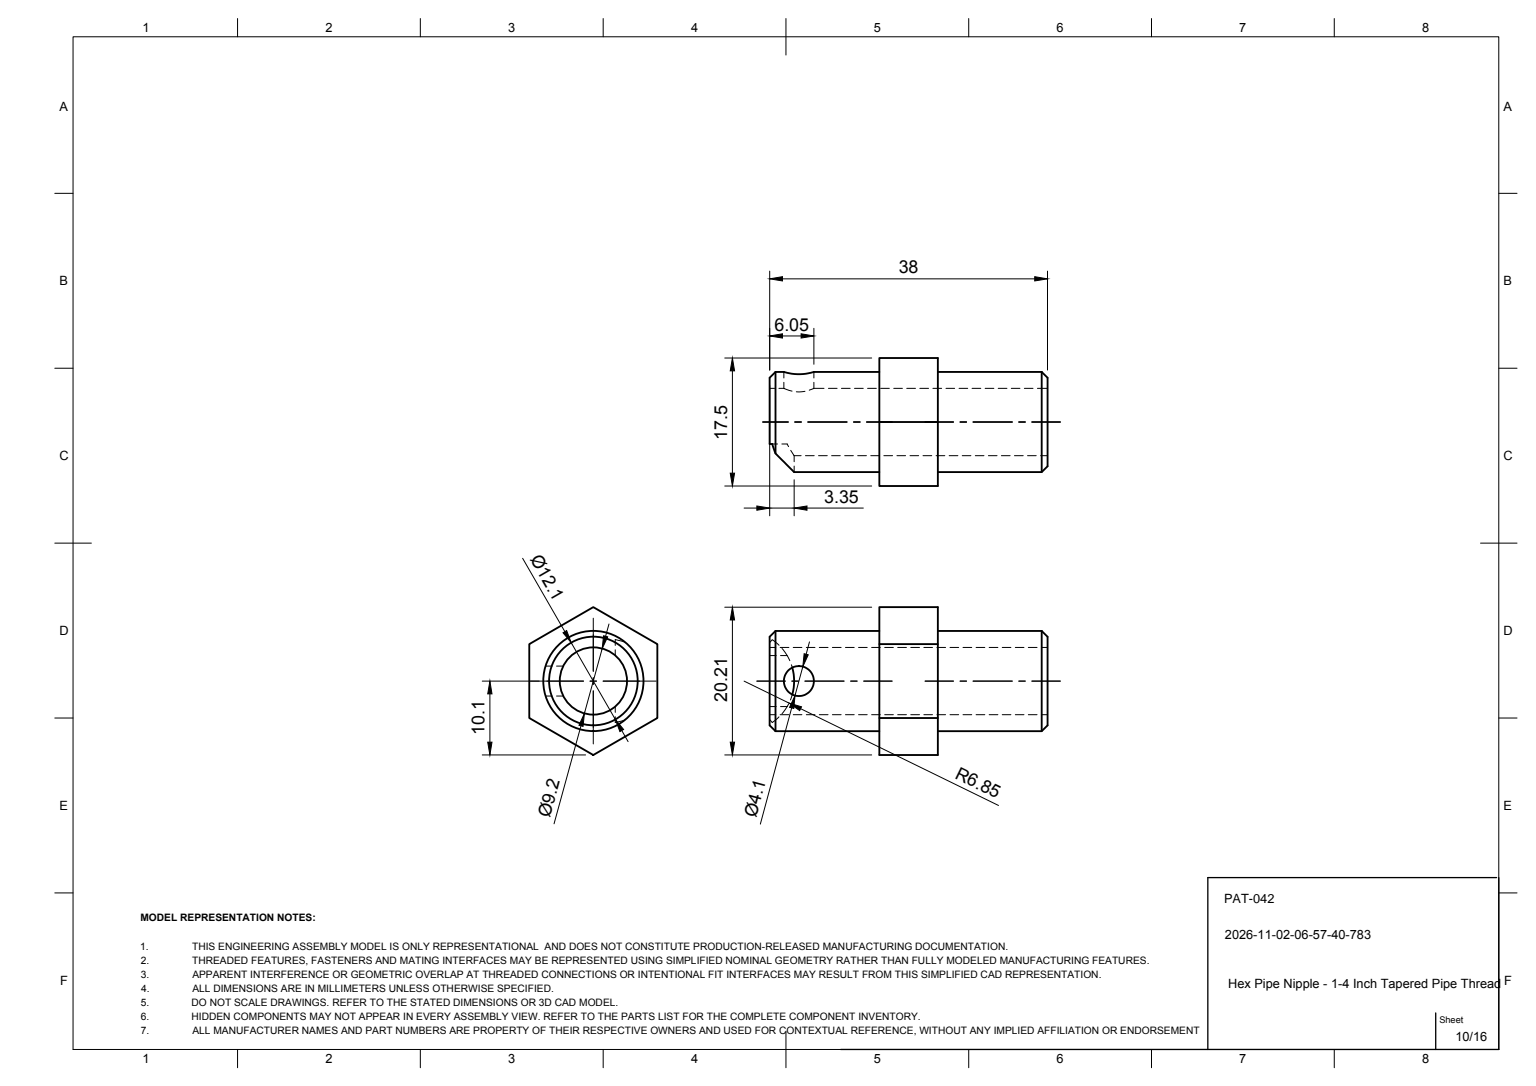
ISO-10303-21;
HEADER;
/* Generated by software containing ST-Developer
 * from STEP Tools, Inc. (www.steptools.com) 
 */

FILE_DESCRIPTION(
/* description */ ('Manifold and mounting hardware'),
/* implementation_level */ '2;1');

FILE_NAME(
/* name */ 'Hex Pipe Nipple - 1-4 Inch Tapered Pipe Thread.step',
/* time_stamp */ '2026-10-28T21:46:49-07:00',
/* author */ (''),
/* organization */ (''),
/* preprocessor_version */ 'ST-DEVELOPER v20.2',
/* originating_system */ 'Autodesk Translation Framework v15.17.0.0',
/* authorisation */ '');

FILE_SCHEMA (('AUTOMOTIVE_DESIGN { 1 0 10303 214 3 1 1 }'));
ENDSEC;

DATA;
#10=MECHANICAL_DESIGN_GEOMETRIC_PRESENTATION_REPRESENTATION('',(#157),#5638);
#118=CONICAL_SURFACE('',#3555,0.645,0.785398163397448);
#129=SHAPE_REPRESENTATION_RELATIONSHIP('SRR','None',#5708,#143);
#143=ADVANCED_BREP_SHAPE_REPRESENTATION('',(#171),#5630);
#157=STYLED_ITEM('',(#5853),#171);
#171=MANIFOLD_SOLID_BREP('Body1',#3147);
#236=FACE_BOUND('',#694,.T.);
#237=FACE_BOUND('',#697,.T.);
#238=FACE_BOUND('',#699,.T.);
#239=FACE_BOUND('',#710,.T.);
#314=CYLINDRICAL_SURFACE('',#3540,0.46);
#315=CYLINDRICAL_SURFACE('',#3552,0.685);
#316=CYLINDRICAL_SURFACE('',#3553,0.685);
#449=FACE_OUTER_BOUND('',#693,.T.);
#450=FACE_OUTER_BOUND('',#695,.T.);
#451=FACE_OUTER_BOUND('',#696,.T.);
#452=FACE_OUTER_BOUND('',#698,.T.);
#453=FACE_OUTER_BOUND('',#700,.T.);
#454=FACE_OUTER_BOUND('',#701,.T.);
#455=FACE_OUTER_BOUND('',#702,.T.);
#456=FACE_OUTER_BOUND('',#703,.T.);
#457=FACE_OUTER_BOUND('',#704,.T.);
#458=FACE_OUTER_BOUND('',#705,.T.);
#459=FACE_OUTER_BOUND('',#706,.T.);
#460=FACE_OUTER_BOUND('',#707,.T.);
#461=FACE_OUTER_BOUND('',#708,.T.);
#462=FACE_OUTER_BOUND('',#709,.T.);
#693=EDGE_LOOP('',(#2574));
#694=EDGE_LOOP('',(#2575));
#695=EDGE_LOOP('',(#2576,#2577,#2578,#2579));
#696=EDGE_LOOP('',(#2580,#2581,#2582,#2583,#2584,#2585));
#697=EDGE_LOOP('',(#2586));
#698=EDGE_LOOP('',(#2587,#2588,#2589,#2590,#2591,#2592));
#699=EDGE_LOOP('',(#2593));
#700=EDGE_LOOP('',(#2594,#2595,#2596,#2597));
#701=EDGE_LOOP('',(#2598,#2599,#2600,#2601));
#702=EDGE_LOOP('',(#2602,#2603,#2604,#2605));
#703=EDGE_LOOP('',(#2606,#2607,#2608,#2609));
#704=EDGE_LOOP('',(#2610,#2611,#2612,#2613));
#705=EDGE_LOOP('',(#2614,#2615,#2616,#2617));
#706=EDGE_LOOP('',(#2618,#2619,#2620,#2621));
#707=EDGE_LOOP('',(#2622,#2623,#2624,#2625));
#708=EDGE_LOOP('',(#2626,#2627,#2628,#2629));
#709=EDGE_LOOP('',(#2630));
#710=EDGE_LOOP('',(#2631));
#861=CIRCLE('',#3538,0.685);
#862=CIRCLE('',#3539,0.46);
#863=CIRCLE('',#3541,0.46);
#864=CIRCLE('',#3543,0.685);
#865=CIRCLE('',#3545,0.685);
#866=CIRCLE('',#3554,0.685);
#867=CIRCLE('',#3556,0.605);
#1058=LINE('',#5290,#1305);
#1059=LINE('',#5294,#1306);
#1060=LINE('',#5296,#1307);
#1061=LINE('',#5298,#1308);
#1062=LINE('',#5300,#1309);
#1063=LINE('',#5302,#1310);
#1064=LINE('',#5303,#1311);
#1065=LINE('',#5309,#1312);
#1066=LINE('',#5311,#1313);
#1067=LINE('',#5313,#1314);
#1068=LINE('',#5315,#1315);
#1069=LINE('',#5317,#1316);
#1070=LINE('',#5318,#1317);
#1071=LINE('',#5322,#1318);
#1072=LINE('',#5323,#1319);
#1073=LINE('',#5325,#1320);
#1074=LINE('',#5327,#1321);
#1075=LINE('',#5329,#1322);
#1076=LINE('',#5331,#1323);
#1077=LINE('',#5334,#1324);
#1078=LINE('',#5338,#1325);
#1079=LINE('',#5342,#1326);
#1305=VECTOR('',#4299,0.46);
#1306=VECTOR('',#4302,1.);
#1307=VECTOR('',#4303,1.);
#1308=VECTOR('',#4304,1.);
#1309=VECTOR('',#4305,1.);
#1310=VECTOR('',#4306,1.);
#1311=VECTOR('',#4307,1.);
#1312=VECTOR('',#4312,1.);
#1313=VECTOR('',#4313,1.);
#1314=VECTOR('',#4314,1.);
#1315=VECTOR('',#4315,1.);
#1316=VECTOR('',#4316,1.);
#1317=VECTOR('',#4317,1.);
#1318=VECTOR('',#4322,1.);
#1319=VECTOR('',#4323,1.);
#1320=VECTOR('',#4326,1.);
#1321=VECTOR('',#4329,1.);
#1322=VECTOR('',#4332,1.);
#1323=VECTOR('',#4335,1.);
#1324=VECTOR('',#4340,0.685);
#1325=VECTOR('',#4345,0.685);
#1326=VECTOR('',#4350,0.645);
#1567=VERTEX_POINT('',#5283);
#1568=VERTEX_POINT('',#5285);
#1569=VERTEX_POINT('',#5288);
#1570=VERTEX_POINT('',#5292);
#1571=VERTEX_POINT('',#5293);
#1572=VERTEX_POINT('',#5295);
#1573=VERTEX_POINT('',#5297);
#1574=VERTEX_POINT('',#5299);
#1575=VERTEX_POINT('',#5301);
#1576=VERTEX_POINT('',#5304);
#1577=VERTEX_POINT('',#5307);
#1578=VERTEX_POINT('',#5308);
#1579=VERTEX_POINT('',#5310);
#1580=VERTEX_POINT('',#5312);
#1581=VERTEX_POINT('',#5314);
#1582=VERTEX_POINT('',#5316);
#1583=VERTEX_POINT('',#5319);
#1584=VERTEX_POINT('',#5336);
#1585=VERTEX_POINT('',#5340);
#1916=EDGE_CURVE('',#1567,#1567,#861,.T.);
#1917=EDGE_CURVE('',#1568,#1568,#862,.T.);
#1918=EDGE_CURVE('',#1569,#1569,#863,.T.);
#1919=EDGE_CURVE('',#1569,#1568,#1058,.T.);
#1920=EDGE_CURVE('',#1570,#1571,#1059,.T.);
#1921=EDGE_CURVE('',#1571,#1572,#1060,.T.);
#1922=EDGE_CURVE('',#1572,#1573,#1061,.T.);
#1923=EDGE_CURVE('',#1573,#1574,#1062,.T.);
#1924=EDGE_CURVE('',#1574,#1575,#1063,.T.);
#1925=EDGE_CURVE('',#1575,#1570,#1064,.T.);
#1926=EDGE_CURVE('',#1576,#1576,#864,.T.);
#1927=EDGE_CURVE('',#1577,#1578,#1065,.T.);
#1928=EDGE_CURVE('',#1578,#1579,#1066,.T.);
#1929=EDGE_CURVE('',#1579,#1580,#1067,.T.);
#1930=EDGE_CURVE('',#1580,#1581,#1068,.T.);
#1931=EDGE_CURVE('',#1581,#1582,#1069,.T.);
#1932=EDGE_CURVE('',#1582,#1577,#1070,.T.);
#1933=EDGE_CURVE('',#1583,#1583,#865,.T.);
#1934=EDGE_CURVE('',#1577,#1571,#1071,.T.);
#1935=EDGE_CURVE('',#1572,#1582,#1072,.T.);
#1936=EDGE_CURVE('',#1573,#1581,#1073,.T.);
#1937=EDGE_CURVE('',#1574,#1580,#1074,.T.);
#1938=EDGE_CURVE('',#1575,#1579,#1075,.T.);
#1939=EDGE_CURVE('',#1570,#1578,#1076,.T.);
#1940=EDGE_CURVE('',#1583,#1567,#1077,.T.);
#1941=EDGE_CURVE('',#1584,#1584,#866,.T.);
#1942=EDGE_CURVE('',#1584,#1576,#1078,.T.);
#1943=EDGE_CURVE('',#1585,#1585,#867,.T.);
#1944=EDGE_CURVE('',#1585,#1584,#1079,.T.);
#2574=ORIENTED_EDGE('',*,*,#1916,.F.);
#2575=ORIENTED_EDGE('',*,*,#1917,.F.);
#2576=ORIENTED_EDGE('',*,*,#1918,.T.);
#2577=ORIENTED_EDGE('',*,*,#1919,.T.);
#2578=ORIENTED_EDGE('',*,*,#1917,.T.);
#2579=ORIENTED_EDGE('',*,*,#1919,.F.);
#2580=ORIENTED_EDGE('',*,*,#1920,.T.);
#2581=ORIENTED_EDGE('',*,*,#1921,.T.);
#2582=ORIENTED_EDGE('',*,*,#1922,.T.);
#2583=ORIENTED_EDGE('',*,*,#1923,.T.);
#2584=ORIENTED_EDGE('',*,*,#1924,.T.);
#2585=ORIENTED_EDGE('',*,*,#1925,.T.);
#2586=ORIENTED_EDGE('',*,*,#1926,.F.);
#2587=ORIENTED_EDGE('',*,*,#1927,.T.);
#2588=ORIENTED_EDGE('',*,*,#1928,.T.);
#2589=ORIENTED_EDGE('',*,*,#1929,.T.);
#2590=ORIENTED_EDGE('',*,*,#1930,.T.);
#2591=ORIENTED_EDGE('',*,*,#1931,.T.);
#2592=ORIENTED_EDGE('',*,*,#1932,.T.);
#2593=ORIENTED_EDGE('',*,*,#1933,.F.);
#2594=ORIENTED_EDGE('',*,*,#1934,.F.);
#2595=ORIENTED_EDGE('',*,*,#1932,.F.);
#2596=ORIENTED_EDGE('',*,*,#1935,.F.);
#2597=ORIENTED_EDGE('',*,*,#1921,.F.);
#2598=ORIENTED_EDGE('',*,*,#1935,.T.);
#2599=ORIENTED_EDGE('',*,*,#1931,.F.);
#2600=ORIENTED_EDGE('',*,*,#1936,.F.);
#2601=ORIENTED_EDGE('',*,*,#1922,.F.);
#2602=ORIENTED_EDGE('',*,*,#1936,.T.);
#2603=ORIENTED_EDGE('',*,*,#1930,.F.);
#2604=ORIENTED_EDGE('',*,*,#1937,.F.);
#2605=ORIENTED_EDGE('',*,*,#1923,.F.);
#2606=ORIENTED_EDGE('',*,*,#1937,.T.);
#2607=ORIENTED_EDGE('',*,*,#1929,.F.);
#2608=ORIENTED_EDGE('',*,*,#1938,.F.);
#2609=ORIENTED_EDGE('',*,*,#1924,.F.);
#2610=ORIENTED_EDGE('',*,*,#1938,.T.);
#2611=ORIENTED_EDGE('',*,*,#1928,.F.);
#2612=ORIENTED_EDGE('',*,*,#1939,.F.);
#2613=ORIENTED_EDGE('',*,*,#1925,.F.);
#2614=ORIENTED_EDGE('',*,*,#1939,.T.);
#2615=ORIENTED_EDGE('',*,*,#1927,.F.);
#2616=ORIENTED_EDGE('',*,*,#1934,.T.);
#2617=ORIENTED_EDGE('',*,*,#1920,.F.);
#2618=ORIENTED_EDGE('',*,*,#1933,.T.);
#2619=ORIENTED_EDGE('',*,*,#1940,.T.);
#2620=ORIENTED_EDGE('',*,*,#1916,.T.);
#2621=ORIENTED_EDGE('',*,*,#1940,.F.);
#2622=ORIENTED_EDGE('',*,*,#1941,.F.);
#2623=ORIENTED_EDGE('',*,*,#1942,.T.);
#2624=ORIENTED_EDGE('',*,*,#1926,.T.);
#2625=ORIENTED_EDGE('',*,*,#1942,.F.);
#2626=ORIENTED_EDGE('',*,*,#1943,.F.);
#2627=ORIENTED_EDGE('',*,*,#1944,.T.);
#2628=ORIENTED_EDGE('',*,*,#1941,.T.);
#2629=ORIENTED_EDGE('',*,*,#1944,.F.);
#2630=ORIENTED_EDGE('',*,*,#1943,.T.);
#2631=ORIENTED_EDGE('',*,*,#1918,.F.);
#2908=PLANE('',#3537);
#2909=PLANE('',#3542);
#2910=PLANE('',#3544);
#2911=PLANE('',#3546);
#2912=PLANE('',#3547);
#2913=PLANE('',#3548);
#2914=PLANE('',#3549);
#2915=PLANE('',#3550);
#2916=PLANE('',#3551);
#2917=PLANE('',#3557);
#3073=ADVANCED_FACE('',(#449,#236),#2908,.T.);
#3074=ADVANCED_FACE('',(#450),#314,.F.);
#3075=ADVANCED_FACE('',(#451,#237),#2909,.F.);
#3076=ADVANCED_FACE('',(#452,#238),#2910,.T.);
#3077=ADVANCED_FACE('',(#453),#2911,.T.);
#3078=ADVANCED_FACE('',(#454),#2912,.T.);
#3079=ADVANCED_FACE('',(#455),#2913,.T.);
#3080=ADVANCED_FACE('',(#456),#2914,.T.);
#3081=ADVANCED_FACE('',(#457),#2915,.T.);
#3082=ADVANCED_FACE('',(#458),#2916,.T.);
#3083=ADVANCED_FACE('',(#459),#315,.T.);
#3084=ADVANCED_FACE('',(#460),#316,.T.);
#3085=ADVANCED_FACE('',(#461),#118,.T.);
#3086=ADVANCED_FACE('',(#462,#239),#2917,.T.);
#3147=CLOSED_SHELL('',(#3073,#3074,#3075,#3076,#3077,#3078,#3079,#3080,
#3081,#3082,#3083,#3084,#3085,#3086));
#3536=AXIS2_PLACEMENT_3D('',#5281,#4287,#4288);
#3537=AXIS2_PLACEMENT_3D('',#5282,#4289,#4290);
#3538=AXIS2_PLACEMENT_3D('',#5284,#4291,#4292);
#3539=AXIS2_PLACEMENT_3D('',#5286,#4293,#4294);
#3540=AXIS2_PLACEMENT_3D('',#5287,#4295,#4296);
#3541=AXIS2_PLACEMENT_3D('',#5289,#4297,#4298);
#3542=AXIS2_PLACEMENT_3D('',#5291,#4300,#4301);
#3543=AXIS2_PLACEMENT_3D('',#5305,#4308,#4309);
#3544=AXIS2_PLACEMENT_3D('',#5306,#4310,#4311);
#3545=AXIS2_PLACEMENT_3D('',#5320,#4318,#4319);
#3546=AXIS2_PLACEMENT_3D('',#5321,#4320,#4321);
#3547=AXIS2_PLACEMENT_3D('',#5324,#4324,#4325);
#3548=AXIS2_PLACEMENT_3D('',#5326,#4327,#4328);
#3549=AXIS2_PLACEMENT_3D('',#5328,#4330,#4331);
#3550=AXIS2_PLACEMENT_3D('',#5330,#4333,#4334);
#3551=AXIS2_PLACEMENT_3D('',#5332,#4336,#4337);
#3552=AXIS2_PLACEMENT_3D('',#5333,#4338,#4339);
#3553=AXIS2_PLACEMENT_3D('',#5335,#4341,#4342);
#3554=AXIS2_PLACEMENT_3D('',#5337,#4343,#4344);
#3555=AXIS2_PLACEMENT_3D('',#5339,#4346,#4347);
#3556=AXIS2_PLACEMENT_3D('',#5341,#4348,#4349);
#3557=AXIS2_PLACEMENT_3D('',#5343,#4351,#4352);
#4287=DIRECTION('axis',(0.,0.,1.));
#4288=DIRECTION('refdir',(1.,0.,0.));
#4289=DIRECTION('center_axis',(1.14015052621434E-31,1.,-1.55447022770527E-24));
#4290=DIRECTION('ref_axis',(-1.,1.10933564796705E-31,5.55111512312579E-17));
#4291=DIRECTION('center_axis',(-1.14015052621434E-31,-1.,1.55447022770527E-24));
#4292=DIRECTION('ref_axis',(1.,0.,0.));
#4293=DIRECTION('center_axis',(1.14015052621434E-31,1.,-1.55447022770527E-24));
#4294=DIRECTION('ref_axis',(1.,0.,0.));
#4295=DIRECTION('center_axis',(0.,-1.,0.));
#4296=DIRECTION('ref_axis',(1.,0.,0.));
#4297=DIRECTION('center_axis',(0.,-1.,0.));
#4298=DIRECTION('ref_axis',(1.,0.,0.));
#4299=DIRECTION('',(0.,1.,0.));
#4300=DIRECTION('center_axis',(0.,1.,0.));
#4301=DIRECTION('ref_axis',(1.,0.,0.));
#4302=DIRECTION('',(-0.5,0.,0.866025403784439));
#4303=DIRECTION('',(-1.,0.,-3.29650746237182E-16));
#4304=DIRECTION('',(-0.5,0.,-0.866025403784439));
#4305=DIRECTION('',(0.5,0.,-0.866025403784438));
#4306=DIRECTION('',(1.,0.,0.));
#4307=DIRECTION('',(0.5,0.,0.866025403784439));
#4308=DIRECTION('center_axis',(0.,-1.,0.));
#4309=DIRECTION('ref_axis',(1.,0.,0.));
#4310=DIRECTION('center_axis',(0.,1.,0.));
#4311=DIRECTION('ref_axis',(1.,0.,0.));
#4312=DIRECTION('',(0.5,0.,-0.866025403784439));
#4313=DIRECTION('',(-0.5,0.,-0.866025403784439));
#4314=DIRECTION('',(-1.,0.,0.));
#4315=DIRECTION('',(-0.5,0.,0.866025403784438));
#4316=DIRECTION('',(0.5,0.,0.866025403784439));
#4317=DIRECTION('',(1.,0.,3.29650746237182E-16));
#4318=DIRECTION('center_axis',(0.,1.,0.));
#4319=DIRECTION('ref_axis',(1.,0.,0.));
#4320=DIRECTION('center_axis',(-3.29650746237182E-16,0.,1.));
#4321=DIRECTION('ref_axis',(1.,0.,3.29650746237182E-16));
#4322=DIRECTION('',(0.,-1.,0.));
#4323=DIRECTION('',(0.,1.,0.));
#4324=DIRECTION('center_axis',(-0.866025403784439,0.,0.5));
#4325=DIRECTION('ref_axis',(0.5,0.,0.866025403784439));
#4326=DIRECTION('',(0.,1.,0.));
#4327=DIRECTION('center_axis',(-0.866025403784439,0.,-0.5));
#4328=DIRECTION('ref_axis',(-0.5,0.,0.866025403784439));
#4329=DIRECTION('',(0.,1.,0.));
#4330=DIRECTION('center_axis',(0.,0.,-1.));
#4331=DIRECTION('ref_axis',(-1.,0.,0.));
#4332=DIRECTION('',(0.,1.,0.));
#4333=DIRECTION('center_axis',(0.866025403784439,0.,-0.5));
#4334=DIRECTION('ref_axis',(-0.5,0.,-0.866025403784439));
#4335=DIRECTION('',(0.,1.,0.));
#4336=DIRECTION('center_axis',(0.866025403784439,0.,0.5));
#4337=DIRECTION('ref_axis',(0.5,0.,-0.866025403784439));
#4338=DIRECTION('center_axis',(0.,-1.,0.));
#4339=DIRECTION('ref_axis',(1.,0.,0.));
#4340=DIRECTION('',(0.,1.,0.));
#4341=DIRECTION('center_axis',(0.,-1.,0.));
#4342=DIRECTION('ref_axis',(1.,0.,0.));
#4343=DIRECTION('center_axis',(0.,-1.,0.));
#4344=DIRECTION('ref_axis',(1.,0.,0.));
#4345=DIRECTION('',(0.,1.,0.));
#4346=DIRECTION('center_axis',(0.,1.,0.));
#4347=DIRECTION('ref_axis',(1.,0.,0.));
#4348=DIRECTION('center_axis',(0.,-1.,0.));
#4349=DIRECTION('ref_axis',(1.,0.,0.));
#4350=DIRECTION('',(-0.707106781186547,0.707106781186548,-8.65956056235493E-17));
#4351=DIRECTION('center_axis',(0.,-1.,0.));
#4352=DIRECTION('ref_axis',(0.,0.,-1.));
#5281=CARTESIAN_POINT('',(0.,0.,0.));
#5282=CARTESIAN_POINT('Origin',(7.91033905045424E-16,1.2,-1.33226762846206E-15));
#5283=CARTESIAN_POINT('',(-0.685,1.2,-8.38883057415937E-17));
#5284=CARTESIAN_POINT('Origin',(0.,1.2,0.));
#5285=CARTESIAN_POINT('',(-0.46,1.2,5.63337527607782E-17));
#5286=CARTESIAN_POINT('Origin',(0.,1.2,0.));
#5287=CARTESIAN_POINT('Origin',(0.,0.,0.));
#5288=CARTESIAN_POINT('',(-0.46,-1.9,-5.63337527607782E-17));
#5289=CARTESIAN_POINT('Origin',(0.,-1.9,0.));
#5290=CARTESIAN_POINT('',(-0.46,0.,-5.63337527607782E-17));
#5291=CARTESIAN_POINT('Origin',(0.,-0.4,0.));
#5292=CARTESIAN_POINT('',(1.01036297108185,-0.4,0.));
#5293=CARTESIAN_POINT('',(0.505181485540923,-0.4,0.875));
#5294=CARTESIAN_POINT('',(0.505181485540923,-0.4,0.875));
#5295=CARTESIAN_POINT('',(-0.505181485540923,-0.4,0.875));
#5296=CARTESIAN_POINT('',(-0.505181485540923,-0.4,0.875));
#5297=CARTESIAN_POINT('',(-1.01036297108185,-0.4,-1.23733777851239E-16));
#5298=CARTESIAN_POINT('',(-1.01036297108185,-0.4,-1.23733777851239E-16));
#5299=CARTESIAN_POINT('',(-0.505181485540922,-0.4,-0.875));
#5300=CARTESIAN_POINT('',(-0.505181485540922,-0.4,-0.875));
#5301=CARTESIAN_POINT('',(0.505181485540923,-0.4,-0.875));
#5302=CARTESIAN_POINT('',(0.505181485540923,-0.4,-0.875));
#5303=CARTESIAN_POINT('',(1.01036297108185,-0.4,0.));
#5304=CARTESIAN_POINT('',(-0.685,-0.4,-8.38883057415937E-17));
#5305=CARTESIAN_POINT('Origin',(0.,-0.4,0.));
#5306=CARTESIAN_POINT('Origin',(0.,0.4,0.));
#5307=CARTESIAN_POINT('',(0.505181485540923,0.4,0.875));
#5308=CARTESIAN_POINT('',(1.01036297108185,0.4,0.));
#5309=CARTESIAN_POINT('',(0.505181485540923,0.4,0.875));
#5310=CARTESIAN_POINT('',(0.505181485540923,0.4,-0.875));
#5311=CARTESIAN_POINT('',(1.01036297108185,0.4,0.));
#5312=CARTESIAN_POINT('',(-0.505181485540922,0.4,-0.875));
#5313=CARTESIAN_POINT('',(0.505181485540923,0.4,-0.875));
#5314=CARTESIAN_POINT('',(-1.01036297108185,0.4,-1.23733777851239E-16));
#5315=CARTESIAN_POINT('',(-0.505181485540922,0.4,-0.875));
#5316=CARTESIAN_POINT('',(-0.505181485540923,0.4,0.875));
#5317=CARTESIAN_POINT('',(-1.01036297108185,0.4,-1.23733777851239E-16));
#5318=CARTESIAN_POINT('',(-0.505181485540923,0.4,0.875));
#5319=CARTESIAN_POINT('',(-0.685,0.4,8.38883057415937E-17));
#5320=CARTESIAN_POINT('Origin',(0.,0.4,0.));
#5321=CARTESIAN_POINT('Origin',(-0.505181485540923,0.,0.875));
#5322=CARTESIAN_POINT('',(0.505181485540923,0.,0.875));
#5323=CARTESIAN_POINT('',(-0.505181485540923,0.,0.875));
#5324=CARTESIAN_POINT('Origin',(-1.01036297108185,0.,-1.23733777851239E-16));
#5325=CARTESIAN_POINT('',(-1.01036297108185,0.,-1.23733777851239E-16));
#5326=CARTESIAN_POINT('Origin',(-0.505181485540922,0.,-0.875));
#5327=CARTESIAN_POINT('',(-0.505181485540922,0.,-0.875));
#5328=CARTESIAN_POINT('Origin',(0.505181485540923,0.,-0.875));
#5329=CARTESIAN_POINT('',(0.505181485540923,0.,-0.875));
#5330=CARTESIAN_POINT('Origin',(1.01036297108185,0.,0.));
#5331=CARTESIAN_POINT('',(1.01036297108185,0.,0.));
#5332=CARTESIAN_POINT('Origin',(0.505181485540923,0.,0.875));
#5333=CARTESIAN_POINT('Origin',(0.,0.,0.));
#5334=CARTESIAN_POINT('',(-0.685,0.,-8.38883057415937E-17));
#5335=CARTESIAN_POINT('Origin',(0.,0.,0.));
#5336=CARTESIAN_POINT('',(-0.685,-1.82,-8.38883057415937E-17));
#5337=CARTESIAN_POINT('Origin',(0.,-1.82,0.));
#5338=CARTESIAN_POINT('',(-0.685,0.,-8.38883057415937E-17));
#5339=CARTESIAN_POINT('Origin',(0.,-1.86,0.));
#5340=CARTESIAN_POINT('',(-0.605,-1.9,-7.40911313484149E-17));
#5341=CARTESIAN_POINT('Origin',(0.,-1.9,0.));
#5342=CARTESIAN_POINT('',(-0.645,-1.86,-7.89897185450043E-17));
#5343=CARTESIAN_POINT('Origin',(0.46,-1.9,0.));
#5613=UNCERTAINTY_MEASURE_WITH_UNIT(LENGTH_MEASURE(0.001),#5639,
'DISTANCE_ACCURACY_VALUE',
'Maximum model space distance between geometric entities at asserted c
onnectivities');
#5621=UNCERTAINTY_MEASURE_WITH_UNIT(LENGTH_MEASURE(0.001),#5639,
'DISTANCE_ACCURACY_VALUE',
'Maximum model space distance between geometric entities at asserted c
onnectivities');
#5630=(
GEOMETRIC_REPRESENTATION_CONTEXT(3)
GLOBAL_UNCERTAINTY_ASSIGNED_CONTEXT((#5613))
GLOBAL_UNIT_ASSIGNED_CONTEXT((#5639,#5641,#5642))
REPRESENTATION_CONTEXT('','3D')
);
#5638=(
GEOMETRIC_REPRESENTATION_CONTEXT(3)
GLOBAL_UNCERTAINTY_ASSIGNED_CONTEXT((#5621))
GLOBAL_UNIT_ASSIGNED_CONTEXT((#5639,#5641,#5642))
REPRESENTATION_CONTEXT('','3D')
);
#5639=(
LENGTH_UNIT()
NAMED_UNIT(*)
SI_UNIT(.CENTI.,.METRE.)
);
#5641=(
NAMED_UNIT(*)
PLANE_ANGLE_UNIT()
SI_UNIT($,.RADIAN.)
);
#5642=(
NAMED_UNIT(*)
SI_UNIT($,.STERADIAN.)
SOLID_ANGLE_UNIT()
);
#5651=SHAPE_DEFINITION_REPRESENTATION(#5667,#5708);
#5667=PRODUCT_DEFINITION_SHAPE('',$,#5725);
#5708=SHAPE_REPRESENTATION('',(#3536),#5630);
#5716=PRODUCT_DEFINITION_CONTEXT('part definition',#5766,'design');
#5725=PRODUCT_DEFINITION('Hex Pipe Nipple - 1-4 Inch Tapered Pipe Thread',
'Hex Pipe Nipple - 1-4 Inch Tapered Pipe Thread',#5741,#5716);
#5741=PRODUCT_DEFINITION_FORMATION('',$,#5776);
#5766=APPLICATION_CONTEXT(
'Core Data for Automotive Mechanical Design Process');
#5767=PRODUCT_CONTEXT('part definition',#5766,'mechanical');
#5776=PRODUCT('Hex Pipe Nipple - 1-4 Inch Tapered Pipe Thread',
'Hex Pipe Nipple - 1-4 Inch Tapered Pipe Thread',
'Hex Pipe Nipple - 1-4 Inch Tapered Pipe Thread',(#5767));
#5847=COLOUR_RGB('Sky Blue',0.24,0.69,0.87);
#5848=FILL_AREA_STYLE_COLOUR('',#5847);
#5849=FILL_AREA_STYLE('',(#5848));
#5850=SURFACE_STYLE_FILL_AREA(#5849);
#5851=SURFACE_SIDE_STYLE('',(#5850));
#5852=SURFACE_STYLE_USAGE(.BOTH.,#5851);
#5853=PRESENTATION_STYLE_ASSIGNMENT((#5852));
ENDSEC;
END-ISO-10303-21;
